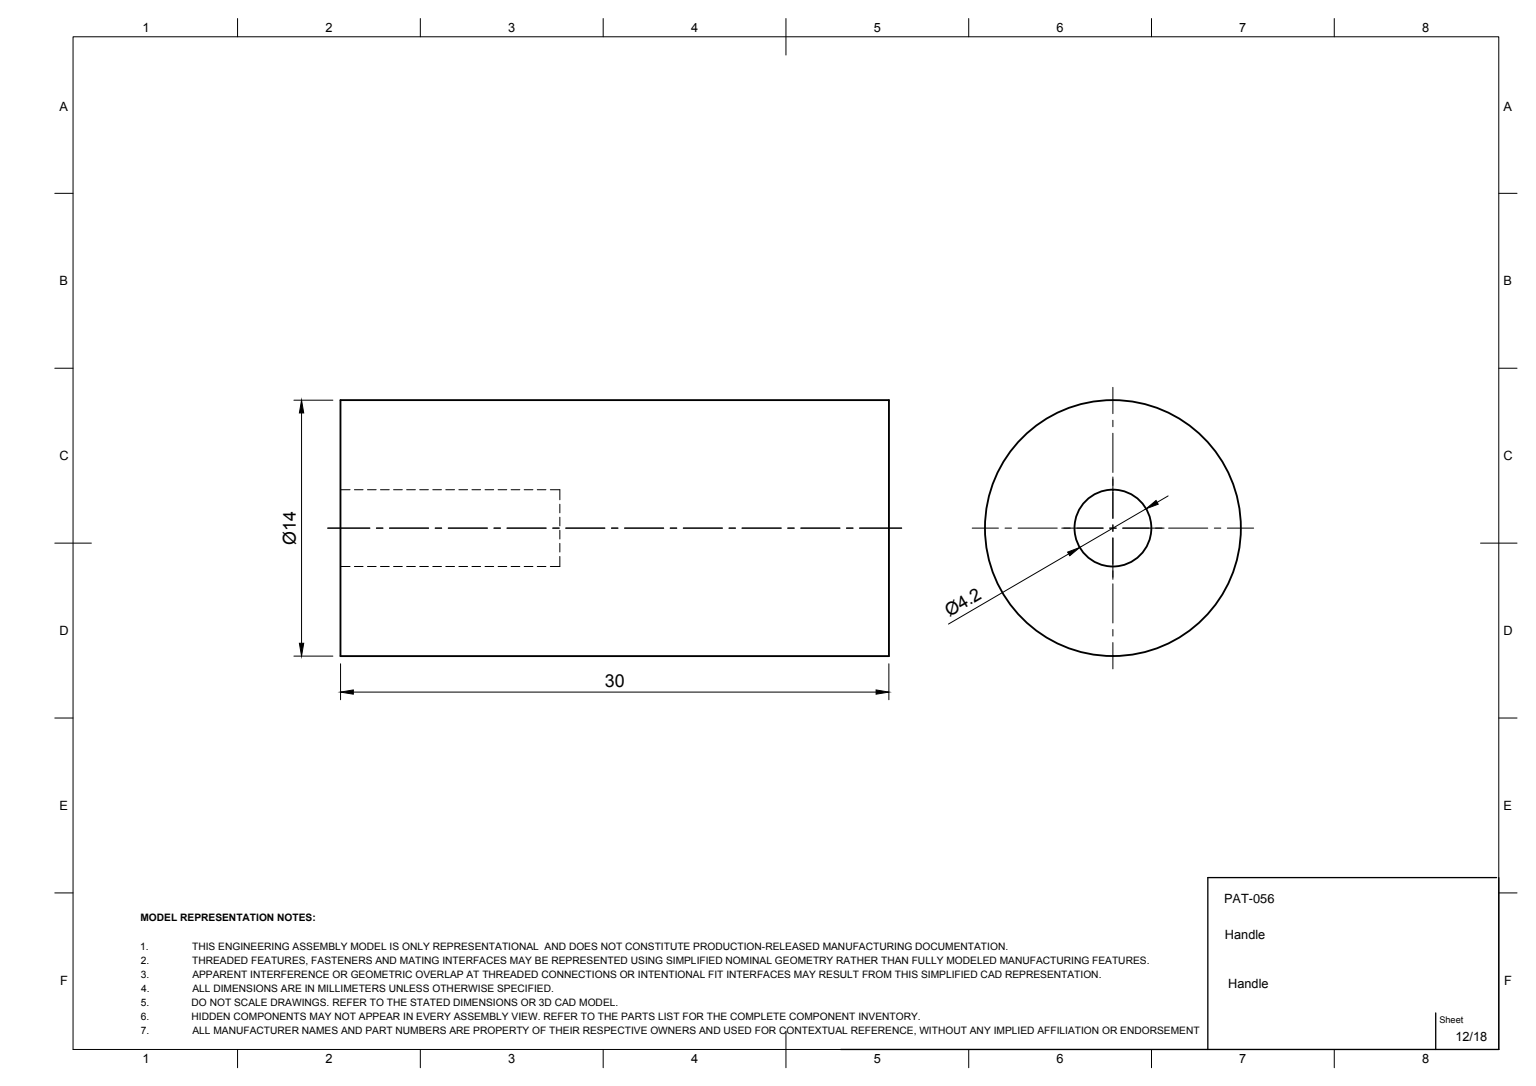
ISO-10303-21;
HEADER;
/* Generated by software containing ST-Developer
 * from STEP Tools, Inc. (www.steptools.com) 
 */

FILE_DESCRIPTION(
/* description */ ('Hook toggle clamp'),
/* implementation_level */ '2;1');

FILE_NAME(
/* name */ 'Handle.step',
/* time_stamp */ '2026-10-27T21:56:56-07:00',
/* author */ (''),
/* organization */ (''),
/* preprocessor_version */ 'ST-DEVELOPER v20.2',
/* originating_system */ 'Autodesk Translation Framework v15.17.0.0',
/* authorisation */ '');

FILE_SCHEMA (('AUTOMOTIVE_DESIGN { 1 0 10303 214 3 1 1 }'));
ENDSEC;

DATA;
#10=MECHANICAL_DESIGN_GEOMETRIC_PRESENTATION_REPRESENTATION('',(#195),#5458);
#161=SHAPE_REPRESENTATION_RELATIONSHIP('SRR','None',#5543,#178);
#178=ADVANCED_BREP_SHAPE_REPRESENTATION('',(#212),#5445);
#195=STYLED_ITEM('',(#5710),#212);
#212=MANIFOLD_SOLID_BREP('Body1',#2976);
#253=FACE_BOUND('',#683,.T.);
#338=PLANE('',#3318);
#339=PLANE('',#3322);
#340=PLANE('',#3323);
#475=FACE_OUTER_BOUND('',#679,.T.);
#476=FACE_OUTER_BOUND('',#680,.T.);
#477=FACE_OUTER_BOUND('',#681,.T.);
#478=FACE_OUTER_BOUND('',#682,.T.);
#479=FACE_OUTER_BOUND('',#684,.T.);
#679=EDGE_LOOP('',(#2389,#2390,#2391,#2392));
#680=EDGE_LOOP('',(#2393));
#681=EDGE_LOOP('',(#2394,#2395,#2396,#2397));
#682=EDGE_LOOP('',(#2398));
#683=EDGE_LOOP('',(#2399));
#684=EDGE_LOOP('',(#2400));
#936=LINE('',#4849,#1173);
#937=LINE('',#4856,#1174);
#1173=VECTOR('',#3934,0.21);
#1174=VECTOR('',#3943,0.7);
#1316=CIRCLE('',#3316,0.21);
#1317=CIRCLE('',#3317,0.21);
#1318=CIRCLE('',#3320,0.7);
#1319=CIRCLE('',#3321,0.7);
#1511=VERTEX_POINT('',#4846);
#1512=VERTEX_POINT('',#4848);
#1513=VERTEX_POINT('',#4853);
#1514=VERTEX_POINT('',#4855);
#1821=EDGE_CURVE('',#1511,#1511,#1316,.T.);
#1822=EDGE_CURVE('',#1511,#1512,#936,.T.);
#1823=EDGE_CURVE('',#1512,#1512,#1317,.T.);
#1824=EDGE_CURVE('',#1513,#1513,#1318,.T.);
#1825=EDGE_CURVE('',#1513,#1514,#937,.T.);
#1826=EDGE_CURVE('',#1514,#1514,#1319,.T.);
#2389=ORIENTED_EDGE('',*,*,#1821,.F.);
#2390=ORIENTED_EDGE('',*,*,#1822,.T.);
#2391=ORIENTED_EDGE('',*,*,#1823,.F.);
#2392=ORIENTED_EDGE('',*,*,#1822,.F.);
#2393=ORIENTED_EDGE('',*,*,#1821,.T.);
#2394=ORIENTED_EDGE('',*,*,#1824,.F.);
#2395=ORIENTED_EDGE('',*,*,#1825,.T.);
#2396=ORIENTED_EDGE('',*,*,#1826,.T.);
#2397=ORIENTED_EDGE('',*,*,#1825,.F.);
#2398=ORIENTED_EDGE('',*,*,#1824,.T.);
#2399=ORIENTED_EDGE('',*,*,#1823,.T.);
#2400=ORIENTED_EDGE('',*,*,#1826,.F.);
#2770=CYLINDRICAL_SURFACE('',#3315,0.21);
#2771=CYLINDRICAL_SURFACE('',#3319,0.7);
#2879=ADVANCED_FACE('',(#475),#2770,.F.);
#2880=ADVANCED_FACE('',(#476),#338,.T.);
#2881=ADVANCED_FACE('',(#477),#2771,.T.);
#2882=ADVANCED_FACE('',(#478,#253),#339,.T.);
#2883=ADVANCED_FACE('',(#479),#340,.F.);
#2976=CLOSED_SHELL('',(#2879,#2880,#2881,#2882,#2883));
#3314=AXIS2_PLACEMENT_3D('',#4844,#3928,#3929);
#3315=AXIS2_PLACEMENT_3D('',#4845,#3930,#3931);
#3316=AXIS2_PLACEMENT_3D('',#4847,#3932,#3933);
#3317=AXIS2_PLACEMENT_3D('',#4850,#3935,#3936);
#3318=AXIS2_PLACEMENT_3D('',#4851,#3937,#3938);
#3319=AXIS2_PLACEMENT_3D('',#4852,#3939,#3940);
#3320=AXIS2_PLACEMENT_3D('',#4854,#3941,#3942);
#3321=AXIS2_PLACEMENT_3D('',#4857,#3944,#3945);
#3322=AXIS2_PLACEMENT_3D('',#4858,#3946,#3947);
#3323=AXIS2_PLACEMENT_3D('',#4859,#3948,#3949);
#3928=DIRECTION('axis',(0.,0.,1.));
#3929=DIRECTION('refdir',(1.,0.,0.));
#3930=DIRECTION('center_axis',(0.,1.,0.));
#3931=DIRECTION('ref_axis',(1.,0.,0.));
#3932=DIRECTION('center_axis',(0.,1.,0.));
#3933=DIRECTION('ref_axis',(1.,0.,0.));
#3934=DIRECTION('',(0.,1.,0.));
#3935=DIRECTION('center_axis',(0.,-1.,0.));
#3936=DIRECTION('ref_axis',(1.,0.,0.));
#3937=DIRECTION('center_axis',(0.,1.,0.));
#3938=DIRECTION('ref_axis',(1.,0.,0.));
#3939=DIRECTION('center_axis',(0.,1.,0.));
#3940=DIRECTION('ref_axis',(1.,0.,0.));
#3941=DIRECTION('center_axis',(0.,1.,0.));
#3942=DIRECTION('ref_axis',(1.,0.,0.));
#3943=DIRECTION('',(0.,-1.,0.));
#3944=DIRECTION('center_axis',(0.,1.,0.));
#3945=DIRECTION('ref_axis',(1.,0.,0.));
#3946=DIRECTION('center_axis',(0.,1.,0.));
#3947=DIRECTION('ref_axis',(1.,0.,0.));
#3948=DIRECTION('center_axis',(0.,1.,0.));
#3949=DIRECTION('ref_axis',(1.,0.,0.));
#4844=CARTESIAN_POINT('',(0.,0.,0.));
#4845=CARTESIAN_POINT('Origin',(0.,-7.7,10.03));
#4846=CARTESIAN_POINT('',(-0.21,-7.7,10.03));
#4847=CARTESIAN_POINT('Origin',(0.,-7.7,10.03));
#4848=CARTESIAN_POINT('',(-0.21,-6.5,10.03));
#4849=CARTESIAN_POINT('',(-0.21,-7.7,10.03));
#4850=CARTESIAN_POINT('Origin',(0.,-6.5,10.03));
#4851=CARTESIAN_POINT('Origin',(0.,-7.7,10.03));
#4852=CARTESIAN_POINT('Origin',(0.,-9.5,10.03));
#4853=CARTESIAN_POINT('',(-0.7,-6.5,10.03));
#4854=CARTESIAN_POINT('Origin',(0.,-6.5,10.03));
#4855=CARTESIAN_POINT('',(-0.7,-9.5,10.03));
#4856=CARTESIAN_POINT('',(-0.7,-9.5,10.03));
#4857=CARTESIAN_POINT('Origin',(0.,-9.5,10.03));
#4858=CARTESIAN_POINT('Origin',(0.,-6.5,10.03));
#4859=CARTESIAN_POINT('Origin',(0.,-9.5,10.03));
#5422=UNCERTAINTY_MEASURE_WITH_UNIT(LENGTH_MEASURE(0.001),#5459,
'DISTANCE_ACCURACY_VALUE',
'Maximum model space distance between geometric entities at asserted c
onnectivities');
#5435=UNCERTAINTY_MEASURE_WITH_UNIT(LENGTH_MEASURE(0.001),#5459,
'DISTANCE_ACCURACY_VALUE',
'Maximum model space distance between geometric entities at asserted c
onnectivities');
#5445=(
GEOMETRIC_REPRESENTATION_CONTEXT(3)
GLOBAL_UNCERTAINTY_ASSIGNED_CONTEXT((#5422))
GLOBAL_UNIT_ASSIGNED_CONTEXT((#5459,#5461,#5462))
REPRESENTATION_CONTEXT('','3D')
);
#5458=(
GEOMETRIC_REPRESENTATION_CONTEXT(3)
GLOBAL_UNCERTAINTY_ASSIGNED_CONTEXT((#5435))
GLOBAL_UNIT_ASSIGNED_CONTEXT((#5459,#5461,#5462))
REPRESENTATION_CONTEXT('','3D')
);
#5459=(
LENGTH_UNIT()
NAMED_UNIT(*)
SI_UNIT(.CENTI.,.METRE.)
);
#5461=(
NAMED_UNIT(*)
PLANE_ANGLE_UNIT()
SI_UNIT($,.RADIAN.)
);
#5462=(
NAMED_UNIT(*)
SI_UNIT($,.STERADIAN.)
SOLID_ANGLE_UNIT()
);
#5472=SHAPE_DEFINITION_REPRESENTATION(#5494,#5543);
#5494=PRODUCT_DEFINITION_SHAPE('',$,#5566);
#5543=SHAPE_REPRESENTATION('',(#3314),#5445);
#5556=PRODUCT_DEFINITION_CONTEXT('part definition',#5624,'design');
#5566=PRODUCT_DEFINITION('Handle','Handle',#5588,#5556);
#5588=PRODUCT_DEFINITION_FORMATION('',$,#5635);
#5624=APPLICATION_CONTEXT(
'Core Data for Automotive Mechanical Design Process');
#5625=PRODUCT_CONTEXT('part definition',#5624,'mechanical');
#5635=PRODUCT('Handle','Handle','Handle',(#5625));
#5704=COLOUR_RGB('Sky Blue',0.24,0.69,0.87);
#5705=FILL_AREA_STYLE_COLOUR('',#5704);
#5706=FILL_AREA_STYLE('',(#5705));
#5707=SURFACE_STYLE_FILL_AREA(#5706);
#5708=SURFACE_SIDE_STYLE('',(#5707));
#5709=SURFACE_STYLE_USAGE(.BOTH.,#5708);
#5710=PRESENTATION_STYLE_ASSIGNMENT((#5709));
ENDSEC;
END-ISO-10303-21;
